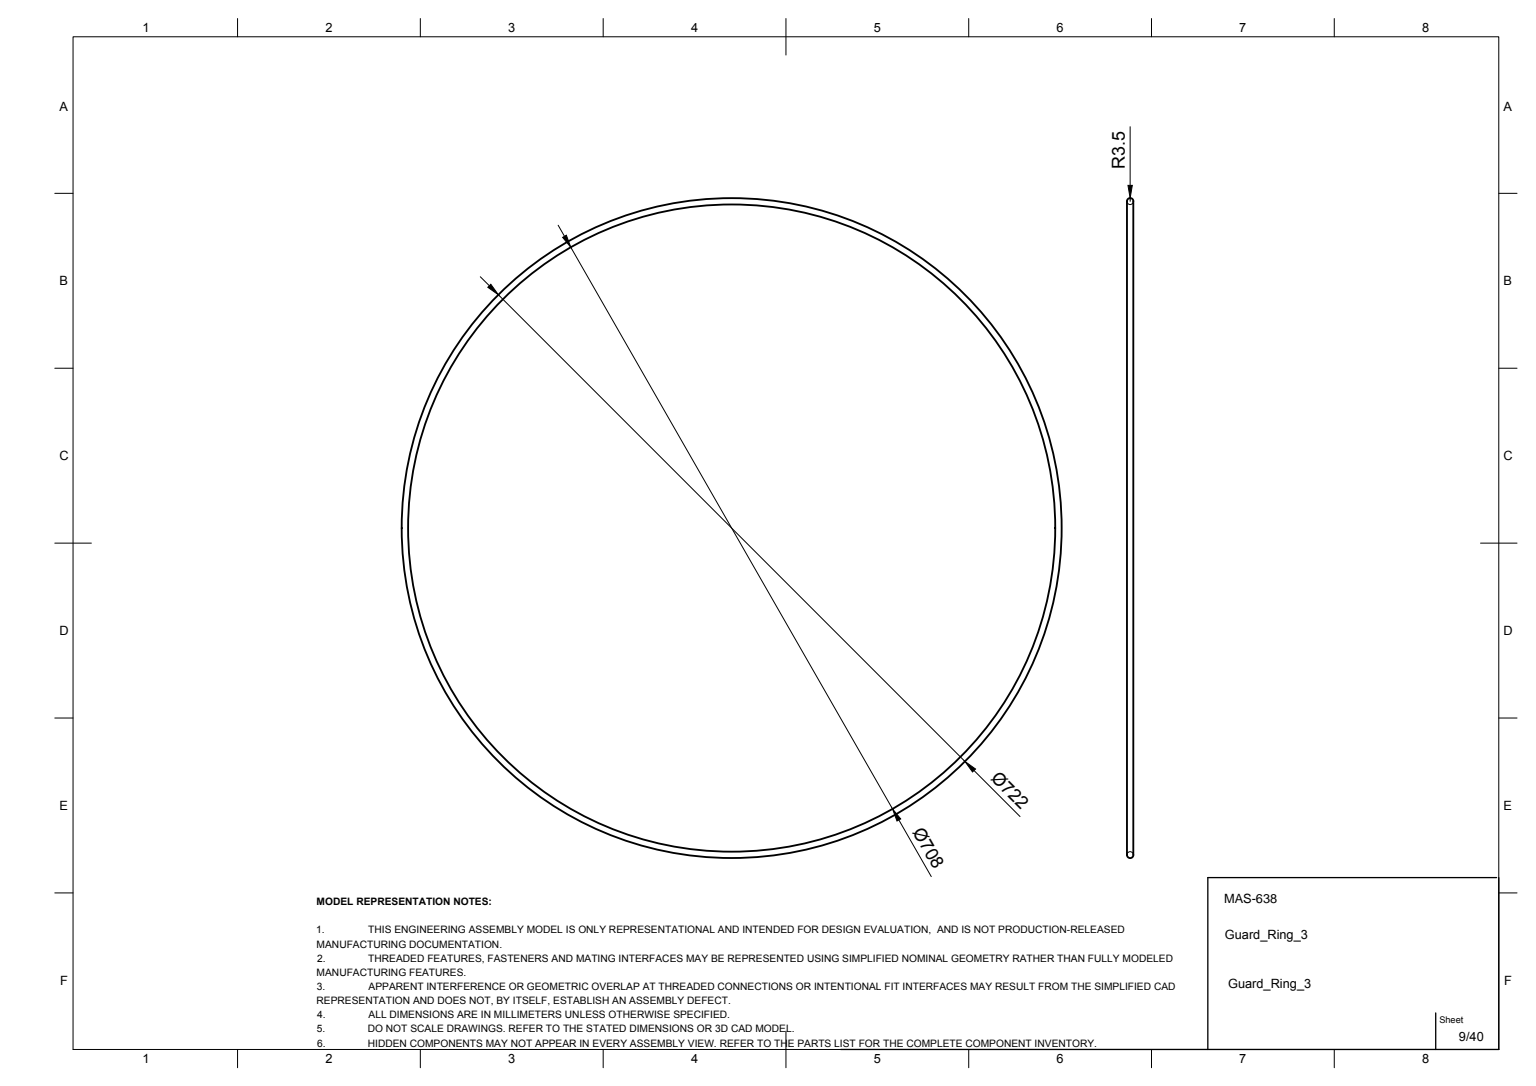
ISO-10303-21;
HEADER;
FILE_DESCRIPTION((''),'2;1');
FILE_NAME('Guard_Ring_3.step','2026-10-09T12:00:21-07:00',(''),(''),'','','');
FILE_SCHEMA (('AUTOMOTIVE_DESIGN { 1 0 10303 214 3 1 1 }'));
ENDSEC;
DATA;
#10=MECHANICAL_DESIGN_GEOMETRIC_PRESENTATION_REPRESENTATION('',(#400),#10334);
#336=SHAPE_REPRESENTATION_RELATIONSHIP('SRR','None',#10452,#368) ;
#368=ADVANCED_BREP_SHAPE_REPRESENTATION('',(#440),#10304) ;
#400=STYLED_ITEM('',(#10631),#440) ;
#440=MANIFOLD_SOLID_BREP('Body1',#3562) ;
#861=FACE_OUTER_BOUND('',#1061,.T.) ;
#1061=EDGE_LOOP('',(#2357,#2358,#2359,#2360)) ;
#1280=CIRCLE('',#3983,0.349999999999999) ;
#1281=CIRCLE('',#3984,35.4) ;
#1515=VERTEX_POINT('',#5663) ;
#1835=EDGE_CURVE('',#1515,#1515,#1280,.T.) ;
#1836=EDGE_CURVE('',#1515,#1515,#1281,.T.) ;
#2357=ORIENTED_EDGE('',*,*,#1835,.F.) ;
#2358=ORIENTED_EDGE('',*,*,#1836,.T.) ;
#2359=ORIENTED_EDGE('',*,*,#1835,.T.) ;
#2360=ORIENTED_EDGE('',*,*,#1836,.F.) ;
#3307=TOROIDAL_SURFACE('',#3982,35.75,0.349999999999999) ;
#3369=ADVANCED_FACE('',(#861),#3307,.T.) ;
#3562=CLOSED_SHELL('',(#3369)) ;
#3981=AXIS2_PLACEMENT_3D('',#5661,#4523,#4524) ;
#3982=AXIS2_PLACEMENT_3D('',#5662,#4525,#4526) ;
#3983=AXIS2_PLACEMENT_3D('',#5664,#4527,#4528) ;
#3984=AXIS2_PLACEMENT_3D('',#5665,#4529,#4530) ;
#4523=DIRECTION('axis',(0.,0.,1.)) ;
#4524=DIRECTION('refdir',(1.,0.,0.)) ;
#4525=DIRECTION('center_axis',(6.42891162084177E-17,1.,1.01883556321148E-16)) ;
#4526=DIRECTION('ref_axis',(-1.,0.,0.)) ;
#4527=DIRECTION('center_axis',(0.,1.01883556321148E-16,-1.)) ;
#4528=DIRECTION('ref_axis',(1.,0.,0.)) ;
#4529=DIRECTION('center_axis',(-6.42891162084177E-17,-1.,-1.01883556321148E-16)) ;
#4530=DIRECTION('ref_axis',(-1.,6.42891162084177E-17,6.55000379205715E-33)) ;
#5661=CARTESIAN_POINT('',(0.,0.,0.)) ;
#5662=CARTESIAN_POINT('Origin',(23.47768801576,63.1830586252741,68.2224337400009)) ;
#5663=CARTESIAN_POINT('',(58.87768801576,63.1830586252741,68.2224337400009)) ;
#5664=CARTESIAN_POINT('Origin',(59.22768801576,63.1830586252741,68.2224337400009)) ;
#5665=CARTESIAN_POINT('Origin',(23.47768801576,63.1830586252741,68.2224337400009)) ;
#10267=UNCERTAINTY_MEASURE_WITH_UNIT(LENGTH_MEASURE(0.001),#10335,
'DISTANCE_ACCURACY_VALUE',
'Maximum model space distance between geometric entities at asserted c
onnectivities') ;
#10297=UNCERTAINTY_MEASURE_WITH_UNIT(LENGTH_MEASURE(0.001),#10335,
'DISTANCE_ACCURACY_VALUE',
'Maximum model space distance between geometric entities at asserted c
onnectivities') ;
#10304=(
GEOMETRIC_REPRESENTATION_CONTEXT(3)
GLOBAL_UNCERTAINTY_ASSIGNED_CONTEXT((#10267))
GLOBAL_UNIT_ASSIGNED_CONTEXT((#10335,#10337,#10338))
REPRESENTATION_CONTEXT('','3D')
) ;
#10334=(
GEOMETRIC_REPRESENTATION_CONTEXT(3)
GLOBAL_UNCERTAINTY_ASSIGNED_CONTEXT((#10297))
GLOBAL_UNIT_ASSIGNED_CONTEXT((#10335,#10337,#10338))
REPRESENTATION_CONTEXT('','3D')
) ;
#10335=(
LENGTH_UNIT()
NAMED_UNIT(*)
SI_UNIT(.CENTI.,.METRE.)
) ;
#10337=(
NAMED_UNIT(*)
PLANE_ANGLE_UNIT()
SI_UNIT($,.RADIAN.)
) ;
#10338=(
NAMED_UNIT(*)
SI_UNIT($,.STERADIAN.)
SOLID_ANGLE_UNIT()
) ;
#10345=SHAPE_DEFINITION_REPRESENTATION(#10381,#10452) ;
#10381=PRODUCT_DEFINITION_SHAPE('',$,#10489) ;
#10452=SHAPE_REPRESENTATION('',(#3981),#10304) ;
#10482=PRODUCT_DEFINITION_CONTEXT('part definition',#10592,'design') ;
#10489=PRODUCT_DEFINITION('Guard_Ring_3','Guard_Ring_3',#10525,#10482) ;
#10525=PRODUCT_DEFINITION_FORMATION('',$,#10600) ;
#10592=APPLICATION_CONTEXT(
'Core Data for Automotive Mechanical Design Process') ;
#10593=PRODUCT_CONTEXT('part definition',#10592,'mechanical') ;
#10600=PRODUCT('Guard_Ring_3','Guard_Ring_3',$,(#10593)) ;
#10631=PRESENTATION_STYLE_ASSIGNMENT((#10635)) ;
#10635=SURFACE_STYLE_USAGE(.BOTH.,#10639) ;
#10639=SURFACE_SIDE_STYLE('',(#10643)) ;
#10643=SURFACE_STYLE_FILL_AREA(#10647) ;
#10647=FILL_AREA_STYLE('Opaque(25,25,25)',(#10651)) ;
#10651=FILL_AREA_STYLE_COLOUR('Opaque(25,25,25)',#10655) ;
#10655=COLOUR_RGB('Opaque(25,25,25)', 0.09019608, 0.27058824, 0.51372549) ;
ENDSEC;
END-ISO-10303-21;
